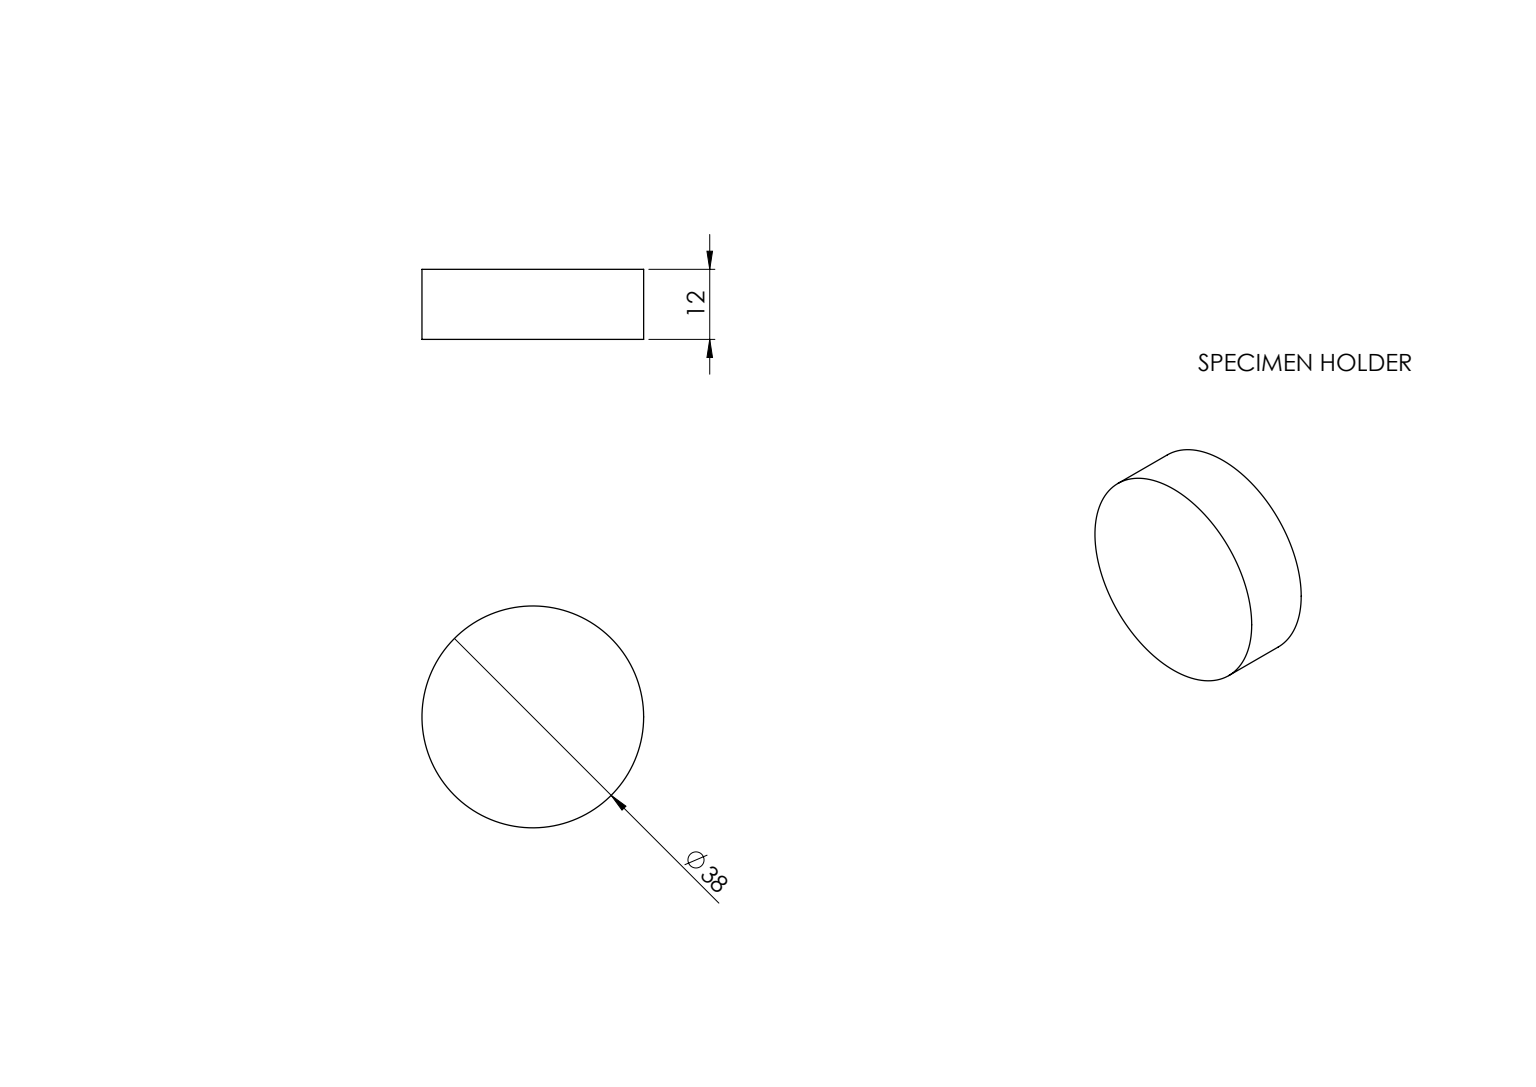
ISO-10303-21;
HEADER;
FILE_DESCRIPTION (('STEP AP214'),
    '1' );
FILE_NAME ('specimen holder.step',
    '2026-10-24T08:20:21',
    ( '' ),
    ( '' ),
    'SwSTEP 2.0',
    'SolidWorks 2026',
    '' );
FILE_SCHEMA (( 'AUTOMOTIVE_DESIGN' ));
ENDSEC;

DATA;
#4=DIRECTION ( 'NONE',  ( -0.000000000000000000, -0.000000000000000000, -1.000000000000000000 ) ) ;
#6=CARTESIAN_POINT ( 'NONE',  ( 0.000000000000000000, 0.000000000000000000, -15.70000000000000284 ) ) ;
#10=ORIENTED_EDGE ( 'NONE', *, *, #2629, .T. ) ;
#15=VERTEX_POINT ( 'NONE', #148 ) ;
#20=AXIS2_PLACEMENT_3D ( 'NONE', #499, #4, #521 ) ;
#29=VECTOR ( 'NONE', #2095, 1000.000000000000000 ) ;
#32=LINE ( 'NONE', #599, #2631 ) ;
#41=PRODUCT_DEFINITION_SHAPE ( 'NONE', 'NONE',  #583 ) ;
#63=ORIENTED_EDGE ( 'NONE', *, *, #1690, .T. ) ;
#78=EDGE_CURVE ( 'NONE', #2558, #3229, #1744, .T. ) ;
#89=CARTESIAN_POINT ( 'NONE',  ( 0.000000000000000000, 0.000000000000000000, -15.70000000000000284 ) ) ;
#97=ORIENTED_EDGE ( 'NONE', *, *, #3095, .F. ) ;
#110=ADVANCED_FACE ( 'NONE', ( #3446, #2287 ), #2899, .F. ) ;
#111=DIRECTION ( 'NONE',  ( -0.000000000000000000, -0.000000000000000000, -1.000000000000000000 ) ) ;
#148=CARTESIAN_POINT ( 'NONE',  ( -1.649999999999999911, 0.000000000000000000, -15.70000000000000284 ) ) ;
#167=ORIENTED_EDGE ( 'NONE', *, *, #1783, .T. ) ;
#177=ADVANCED_FACE ( 'NONE', ( #484 ), #3479, .T. ) ;
#181=FACE_OUTER_BOUND ( 'NONE', #2792, .T. ) ;
#199=PRODUCT_DEFINITION_CONTEXT ( 'detailed design', #1821, 'design' ) ;
#200=DIRECTION ( 'NONE',  ( 0.000000000000000000, 0.000000000000000000, 1.000000000000000000 ) ) ;
#203=MECHANICAL_DESIGN_GEOMETRIC_PRESENTATION_REPRESENTATION('',(#1878),#378);
#213=AXIS2_PLACEMENT_3D ( 'NONE', #1985, #1430, #779 ) ;
#251=CIRCLE ( 'NONE', #760, 18.99999999999999645 ) ;
#263=AXIS2_PLACEMENT_3D ( 'NONE', #1547, #656, #1261 ) ;
#268=( LENGTH_UNIT ( ) NAMED_UNIT ( * ) SI_UNIT ( .MILLI., .METRE. ) );
#280=DIRECTION ( 'NONE',  ( -0.000000000000000000, -0.000000000000000000, -1.000000000000000000 ) ) ;
#286=FACE_OUTER_BOUND ( 'NONE', #2486, .T. ) ;
#345=DIRECTION ( 'NONE',  ( 0.000000000000000000, 0.000000000000000000, 1.000000000000000000 ) ) ;
#348=DIRECTION ( 'NONE',  ( -0.000000000000000000, -0.000000000000000000, -1.000000000000000000 ) ) ;
#370=EDGE_LOOP ( 'NONE', ( #10, #1130 ) ) ;
#378=( GEOMETRIC_REPRESENTATION_CONTEXT ( 3 ) GLOBAL_UNCERTAINTY_ASSIGNED_CONTEXT ( ( #3167 ) ) GLOBAL_UNIT_ASSIGNED_CONTEXT ( ( #1308, #1913, #2493 ) ) REPRESENTATION_CONTEXT ( 'NONE', 'WORKASPACE' ) );
#387=DIRECTION ( 'NONE',  ( -0.000000000000000000, -0.000000000000000000, -1.000000000000000000 ) ) ;
#412=LINE ( 'NONE', #3056, #2644 ) ;
#418=APPLICATION_CONTEXT ( 'automotive_design' ) ;
#427=VERTEX_POINT ( 'NONE', #2778 ) ;
#432=DIRECTION ( 'NONE',  ( -0.000000000000000000, -0.000000000000000000, -1.000000000000000000 ) ) ;
#437=EDGE_CURVE ( 'NONE', #427, #715, #600, .T. ) ;
#445=ORIENTED_EDGE ( 'NONE', *, *, #866, .T. ) ;
#448=CARTESIAN_POINT ( 'NONE',  ( 0.000000000000000000, 0.000000000000000000, -15.70000000000000284 ) ) ;
#461=EDGE_CURVE ( 'NONE', #2373, #2385, #1905, .T. ) ;
#479=ORIENTED_EDGE ( 'NONE', *, *, #638, .F. ) ;
#481=DIRECTION ( 'NONE',  ( 0.000000000000000000, 0.000000000000000000, 1.000000000000000000 ) ) ;
#484=FACE_OUTER_BOUND ( 'NONE', #2820, .T. ) ;
#485=DIRECTION ( 'NONE',  ( -0.000000000000000000, -0.000000000000000000, -1.000000000000000000 ) ) ;
#499=CARTESIAN_POINT ( 'NONE',  ( 0.000000000000000000, 0.000000000000000000, -8.000000000000000000 ) ) ;
#510=DIRECTION ( 'NONE',  ( -0.000000000000000000, -0.000000000000000000, -1.000000000000000000 ) ) ;
#514=AXIS2_PLACEMENT_3D ( 'NONE', #1091, #878, #2301 ) ;
#521=DIRECTION ( 'NONE',  ( -1.000000000000000000, 0.000000000000000000, 0.000000000000000000 ) ) ;
#533=PRODUCT_DEFINITION_FORMATION_WITH_SPECIFIED_SOURCE ( 'ANY', '', #1906, .NOT_KNOWN. ) ;
#544=CARTESIAN_POINT ( 'NONE',  ( 0.000000000000000000, 0.000000000000000000, -8.000000000000000000 ) ) ;
#545=FILL_AREA_STYLE ('',( #2106 ) ) ;
#551=FACE_OUTER_BOUND ( 'NONE', #1433, .T. ) ;
#574=CARTESIAN_POINT ( 'NONE',  ( 0.000000000000000000, 0.000000000000000000, -14.99999999999999645 ) ) ;
#579=ORIENTED_EDGE ( 'NONE', *, *, #2275, .F. ) ;
#583=PRODUCT_DEFINITION ( 'UNKNOWN', '', #533, #199 ) ;
#592=ORIENTED_EDGE ( 'NONE', *, *, #78, .T. ) ;
#594=ORIENTED_EDGE ( 'NONE', *, *, #638, .T. ) ;
#599=CARTESIAN_POINT ( 'NONE',  ( -1.999999999999999112, 0.000000000000000000, -20.00000000000000000 ) ) ;
#600=CIRCLE ( 'NONE', #3082, 1.999999999999998224 ) ;
#611=VERTEX_POINT ( 'NONE', #2374 ) ;
#629=CARTESIAN_POINT ( 'NONE',  ( 0.000000000000000000, 0.000000000000000000, -20.00000000000000000 ) ) ;
#638=EDGE_CURVE ( 'NONE', #15, #2226, #783, .T. ) ;
#656=DIRECTION ( 'NONE',  ( 0.000000000000000000, 0.000000000000000000, 1.000000000000000000 ) ) ;
#674=DIRECTION ( 'NONE',  ( 0.8571673007021117785, 1.049727191138617956E-16, -0.5150380749100550437 ) ) ;
#682=DIRECTION ( 'NONE',  ( -1.000000000000000000, 0.000000000000000000, 0.000000000000000000 ) ) ;
#715=VERTEX_POINT ( 'NONE', #2469 ) ;
#760=AXIS2_PLACEMENT_3D ( 'NONE', #544, #883, #2067 ) ;
#767=CARTESIAN_POINT ( 'NONE',  ( -1.649999999999999245, 0.000000000000000000, -20.00000000000000000 ) ) ;
#770=AXIS2_PLACEMENT_3D ( 'NONE', #3342, #3320, #1841 ) ;
#771=AXIS2_PLACEMENT_3D ( 'NONE', #1959, #2015, #3203 ) ;
#775=DIRECTION ( 'NONE',  ( 1.000000000000000000, 0.000000000000000000, 0.000000000000000000 ) ) ;
#776=ADVANCED_FACE ( 'NONE', ( #1341 ), #3638, .F. ) ;
#779=DIRECTION ( 'NONE',  ( 1.000000000000000000, 0.000000000000000000, -0.000000000000000000 ) ) ;
#783=CIRCLE ( 'NONE', #3389, 1.649999999999999911 ) ;
#784=PRODUCT_CONTEXT ( 'NONE', #418, 'mechanical' ) ;
#797=DIRECTION ( 'NONE',  ( 0.000000000000000000, 0.000000000000000000, 1.000000000000000000 ) ) ;
#805=ORIENTED_EDGE ( 'NONE', *, *, #3212, .T. ) ;
#816=CARTESIAN_POINT ( 'NONE',  ( 0.000000000000000000, 0.000000000000000000, -8.000000000000000000 ) ) ;
#820=CARTESIAN_POINT ( 'NONE',  ( 0.000000000000000000, 0.000000000000000000, 0.000000000000000000 ) ) ;
#842=LINE ( 'NONE', #2086, #1695 ) ;
#843=PRESENTATION_STYLE_ASSIGNMENT (( #2655 ) ) ;
#863=DIRECTION ( 'NONE',  ( -1.000000000000000000, 0.000000000000000000, 0.000000000000000000 ) ) ;
#866=EDGE_CURVE ( 'NONE', #2558, #1368, #412, .T. ) ;
#875=DIRECTION ( 'NONE',  ( 1.000000000000000000, 0.000000000000000000, 0.000000000000000000 ) ) ;
#877=FACE_OUTER_BOUND ( 'NONE', #3535, .T. ) ;
#878=DIRECTION ( 'NONE',  ( -0.000000000000000000, -0.000000000000000000, -1.000000000000000000 ) ) ;
#883=DIRECTION ( 'NONE',  ( 0.000000000000000000, 0.000000000000000000, 1.000000000000000000 ) ) ;
#884=( LENGTH_UNIT ( ) NAMED_UNIT ( * ) SI_UNIT ( .MILLI., .METRE. ) );
#908=( GEOMETRIC_REPRESENTATION_CONTEXT ( 3 ) GLOBAL_UNCERTAINTY_ASSIGNED_CONTEXT ( ( #3619 ) ) GLOBAL_UNIT_ASSIGNED_CONTEXT ( ( #884, #1793, #924 ) ) REPRESENTATION_CONTEXT ( 'NONE', 'WORKASPACE' ) );
#921=ORIENTED_EDGE ( 'NONE', *, *, #437, .T. ) ;
#924=( NAMED_UNIT ( * ) SI_UNIT ( $, .STERADIAN. ) SOLID_ANGLE_UNIT ( ) );
#928=CARTESIAN_POINT ( 'NONE',  ( -1.649999999999998579, 0.000000000000000000, -14.99999999999999645 ) ) ;
#957=DIRECTION ( 'NONE',  ( -0.000000000000000000, -0.000000000000000000, -1.000000000000000000 ) ) ;
#961=SHAPE_REPRESENTATION ( 'specimen holder', ( #2207 ), #908 ) ;
#978=CARTESIAN_POINT ( 'NONE',  ( 0.000000000000000000, 0.000000000000000000, -20.00000000000000000 ) ) ;
#979=CARTESIAN_POINT ( 'NONE',  ( 1.999999999999999112, 2.449293598294705428E-16, -20.00000000000000000 ) ) ;
#992=DIRECTION ( 'NONE',  ( -0.000000000000000000, -0.000000000000000000, -1.000000000000000000 ) ) ;
#1030=ORIENTED_EDGE ( 'NONE', *, *, #3165, .T. ) ;
#1033=DIRECTION ( 'NONE',  ( -0.000000000000000000, -0.000000000000000000, -1.000000000000000000 ) ) ;
#1056=DIRECTION ( 'NONE',  ( -1.000000000000000000, 0.000000000000000000, 0.000000000000000000 ) ) ;
#1067=CARTESIAN_POINT ( 'NONE',  ( 0.000000000000000000, 0.000000000000000000, -14.99999999999999645 ) ) ;
#1089=EDGE_LOOP ( 'NONE', ( #2639, #1113, #2464, #921 ) ) ;
#1091=CARTESIAN_POINT ( 'NONE',  ( 0.000000000000000000, 0.000000000000000000, -15.70000000000000284 ) ) ;
#1105=VERTEX_POINT ( 'NONE', #2333 ) ;
#1113=ORIENTED_EDGE ( 'NONE', *, *, #2629, .F. ) ;
#1130=ORIENTED_EDGE ( 'NONE', *, *, #461, .T. ) ;
#1144=ADVANCED_FACE ( 'NONE', ( #3825 ), #2279, .T. ) ;
#1176=ORIENTED_EDGE ( 'NONE', *, *, #437, .F. ) ;
#1181=DIRECTION ( 'NONE',  ( -0.000000000000000000, -0.000000000000000000, -1.000000000000000000 ) ) ;
#1229=CLOSED_SHELL ( 'NONE', ( #776, #1258, #1235, #177, #1944, #1144, #2674, #3048, #1994, #110, #2461 ) ) ;
#1230=DIRECTION ( 'NONE',  ( -1.000000000000000000, 0.000000000000000000, 0.000000000000000000 ) ) ;
#1235=ADVANCED_FACE ( 'NONE', ( #877 ), #2964, .F. ) ;
#1239=DIRECTION ( 'NONE',  ( -1.000000000000000000, 0.000000000000000000, 0.000000000000000000 ) ) ;
#1258=ADVANCED_FACE ( 'NONE', ( #2744 ), #1594, .F. ) ;
#1261=DIRECTION ( 'NONE',  ( 1.000000000000000000, 0.000000000000000000, -0.000000000000000000 ) ) ;
#1274=EDGE_CURVE ( 'NONE', #2771, #611, #3236, .T. ) ;
#1308=( LENGTH_UNIT ( ) NAMED_UNIT ( * ) SI_UNIT ( .MILLI., .METRE. ) );
#1318=ORIENTED_EDGE ( 'NONE', *, *, #3095, .T. ) ;
#1341=FACE_OUTER_BOUND ( 'NONE', #3463, .T. ) ;
#1368=VERTEX_POINT ( 'NONE', #2293 ) ;
#1370=PLANE ( 'NONE',  #263 ) ;
#1387=CIRCLE ( 'NONE', #3557, 18.99999999999999645 ) ;
#1393=CIRCLE ( 'NONE', #2132, 2.000000000000000000 ) ;
#1394=DIRECTION ( 'NONE',  ( 1.000000000000000000, 0.000000000000000000, 0.000000000000000000 ) ) ;
#1418=ORIENTED_EDGE ( 'NONE', *, *, #2998, .T. ) ;
#1430=DIRECTION ( 'NONE',  ( 0.000000000000000000, 0.000000000000000000, 1.000000000000000000 ) ) ;
#1433=EDGE_LOOP ( 'NONE', ( #2166, #592, #1418 ) ) ;
#1442=EDGE_LOOP ( 'NONE', ( #1318, #2099 ) ) ;
#1448=CIRCLE ( 'NONE', #3371, 18.99999999999999645 ) ;
#1489=EDGE_CURVE ( 'NONE', #1105, #3089, #842, .T. ) ;
#1497=ORIENTED_EDGE ( 'NONE', *, *, #3426, .F. ) ;
#1503=CIRCLE ( 'NONE', #2570, 18.99999999999999645 ) ;
#1507=DIRECTION ( 'NONE',  ( -0.000000000000000000, -0.000000000000000000, -1.000000000000000000 ) ) ;
#1533=EDGE_CURVE ( 'NONE', #2771, #1105, #251, .T. ) ;
#1547=CARTESIAN_POINT ( 'NONE',  ( 0.000000000000000000, 0.000000000000000000, -20.00000000000000000 ) ) ;
#1549=DIRECTION ( 'NONE',  ( -1.000000000000000000, 0.000000000000000000, 0.000000000000000000 ) ) ;
#1580=DIRECTION ( 'NONE',  ( -1.000000000000000000, 0.000000000000000000, 0.000000000000000000 ) ) ;
#1594=CYLINDRICAL_SURFACE ( 'NONE', #1652, 1.649999999999999245 ) ;
#1611=SHAPE_DEFINITION_REPRESENTATION ( #41, #961 ) ;
#1625=CIRCLE ( 'NONE', #3802, 1.649999999999998579 ) ;
#1652=AXIS2_PLACEMENT_3D ( 'NONE', #2785, #111, #2351 ) ;
#1690=EDGE_CURVE ( 'NONE', #2373, #715, #3622, .T. ) ;
#1695=VECTOR ( 'NONE', #3815, 1000.000000000000000 ) ;
#1735=SURFACE_SIDE_STYLE ('',( #3799 ) ) ;
#1744=LINE ( 'NONE', #2916, #2484 ) ;
#1762=CARTESIAN_POINT ( 'NONE',  ( 18.99999999999999645, 2.326828918379970576E-15, -8.000000000000000000 ) ) ;
#1765=CIRCLE ( 'NONE', #2574, 1.649999999999998579 ) ;
#1783=EDGE_CURVE ( 'NONE', #1368, #3229, #1625, .T. ) ;
#1793=( NAMED_UNIT ( * ) PLANE_ANGLE_UNIT ( ) SI_UNIT ( $, .RADIAN. ) );
#1797=ORIENTED_EDGE ( 'NONE', *, *, #461, .F. ) ;
#1821=APPLICATION_CONTEXT ( 'automotive_design' ) ;
#1841=DIRECTION ( 'NONE',  ( -1.000000000000000000, 0.000000000000000000, 0.000000000000000000 ) ) ;
#1845=CARTESIAN_POINT ( 'NONE',  ( 0.000000000000000000, 0.000000000000000000, -20.00000000000000000 ) ) ;
#1878=STYLED_ITEM('',(#3888),#3238);
#1894=COLOUR_RGB ( '',0.8941176470588234615, 0.8941176470588234615, 0.8941176470588234615 ) ;
#1905=CIRCLE ( 'NONE', #3773, 2.000000000000000000 ) ;
#1906=PRODUCT ( 'specimen holder', 'specimen holder', '', ( #784 ) ) ;
#1913=( NAMED_UNIT ( * ) PLANE_ANGLE_UNIT ( ) SI_UNIT ( $, .RADIAN. ) );
#1934=ORIENTED_EDGE ( 'NONE', *, *, #2178, .T. ) ;
#1944=ADVANCED_FACE ( 'NONE', ( #286 ), #2669, .T. ) ;
#1956=ORIENTED_EDGE ( 'NONE', *, *, #2275, .T. ) ;
#1959=CARTESIAN_POINT ( 'NONE',  ( 0.000000000000000000, 0.000000000000000000, -14.99999999999999645 ) ) ;
#1985=CARTESIAN_POINT ( 'NONE',  ( 1.649999999999999911, 0.000000000000000000, -15.70000000000000284 ) ) ;
#1994=ADVANCED_FACE ( 'NONE', ( #3635 ), #3325, .F. ) ;
#2002=DIRECTION ( 'NONE',  ( -0.000000000000000000, -0.000000000000000000, -1.000000000000000000 ) ) ;
#2008=VECTOR ( 'NONE', #3163, 1000.000000000000000 ) ;
#2015=DIRECTION ( 'NONE',  ( -0.000000000000000000, -0.000000000000000000, -1.000000000000000000 ) ) ;
#2055=ORIENTED_EDGE ( 'NONE', *, *, #1274, .F. ) ;
#2067=DIRECTION ( 'NONE',  ( 1.000000000000000000, 0.000000000000000000, 0.000000000000000000 ) ) ;
#2078=CARTESIAN_POINT ( 'NONE',  ( 2.000000000000000000, 2.449293598294706414E-16, -15.70000000000000284 ) ) ;
#2085=DIRECTION ( 'NONE',  ( -0.000000000000000000, -0.000000000000000000, -1.000000000000000000 ) ) ;
#2086=CARTESIAN_POINT ( 'NONE',  ( -18.99999999999999645, 0.000000000000000000, -8.000000000000000000 ) ) ;
#2087=( NAMED_UNIT ( * ) PLANE_ANGLE_UNIT ( ) SI_UNIT ( $, .RADIAN. ) );
#2095=DIRECTION ( 'NONE',  ( -0.000000000000000000, -0.000000000000000000, -1.000000000000000000 ) ) ;
#2099=ORIENTED_EDGE ( 'NONE', *, *, #1533, .T. ) ;
#2106=FILL_AREA_STYLE_COLOUR ( '', #1894 ) ;
#2126=CARTESIAN_POINT ( 'NONE',  ( 1.649999999999999245, 2.020667218593132015E-16, -20.00000000000000000 ) ) ;
#2130=CIRCLE ( 'NONE', #2628, 1.999999999999998224 ) ;
#2132=AXIS2_PLACEMENT_3D ( 'NONE', #448, #387, #1580 ) ;
#2141=STYLED_ITEM ( 'NONE', ( #843 ), #2739 ) ;
#2166=ORIENTED_EDGE ( 'NONE', *, *, #866, .F. ) ;
#2178=EDGE_CURVE ( 'NONE', #611, #3089, #1503, .T. ) ;
#2188=ORIENTED_EDGE ( 'NONE', *, *, #1533, .F. ) ;
#2205=EDGE_LOOP ( 'NONE', ( #479, #579 ) ) ;
#2207=AXIS2_PLACEMENT_3D ( 'NONE', #820, #2246, #3194 ) ;
#2226=VERTEX_POINT ( 'NONE', #2483 ) ;
#2246=DIRECTION ( 'NONE',  ( 0.000000000000000000, 0.000000000000000000, 1.000000000000000000 ) ) ;
#2275=EDGE_CURVE ( 'NONE', #2226, #15, #2504, .T. ) ;
#2276=UNCERTAINTY_MEASURE_WITH_UNIT (LENGTH_MEASURE( 1.000000000000000082E-05 ), #268, 'distance_accuracy_value', 'NONE');
#2279=PLANE ( 'NONE',  #2586 ) ;
#2287=FACE_OUTER_BOUND ( 'NONE', #370, .T. ) ;
#2293=CARTESIAN_POINT ( 'NONE',  ( 1.649999999999998579, 2.020667218593131029E-16, -14.99999999999999645 ) ) ;
#2301=DIRECTION ( 'NONE',  ( -1.000000000000000000, 0.000000000000000000, 0.000000000000000000 ) ) ;
#2333=CARTESIAN_POINT ( 'NONE',  ( -18.99999999999999645, 0.000000000000000000, -8.000000000000000000 ) ) ;
#2351=DIRECTION ( 'NONE',  ( -1.000000000000000000, 0.000000000000000000, 0.000000000000000000 ) ) ;
#2353=EDGE_CURVE ( 'NONE', #715, #427, #2130, .T. ) ;
#2355=ORIENTED_EDGE ( 'NONE', *, *, #1274, .T. ) ;
#2364=ORIENTED_EDGE ( 'NONE', *, *, #1489, .F. ) ;
#2373=VERTEX_POINT ( 'NONE', #2078 ) ;
#2374=CARTESIAN_POINT ( 'NONE',  ( 18.99999999999999645, 2.326828918379970576E-15, -20.00000000000000000 ) ) ;
#2385=VERTEX_POINT ( 'NONE', #3296 ) ;
#2400=SHAPE_REPRESENTATION_RELATIONSHIP ( 'NONE' , 'NONE' ,  #961, #2739 ) ;
#2411=CARTESIAN_POINT ( 'NONE',  ( 18.99999999999999645, 2.326828918379970576E-15, -8.000000000000000000 ) ) ;
#2461=ADVANCED_FACE ( 'NONE', ( #3259 ), #3013, .F. ) ;
#2464=ORIENTED_EDGE ( 'NONE', *, *, #2468, .T. ) ;
#2468=EDGE_CURVE ( 'NONE', #2385, #427, #32, .T. ) ;
#2469=CARTESIAN_POINT ( 'NONE',  ( 1.999999999999998224, 2.449293598294704935E-16, -20.00000000000000355 ) ) ;
#2483=CARTESIAN_POINT ( 'NONE',  ( 1.649999999999999911, 2.020667218593133001E-16, -15.70000000000000284 ) ) ;
#2484=VECTOR ( 'NONE', #2567, 1000.000000000000000 ) ;
#2486=EDGE_LOOP ( 'NONE', ( #2055, #97, #3119, #805 ) ) ;
#2493=( NAMED_UNIT ( * ) SI_UNIT ( $, .STERADIAN. ) SOLID_ANGLE_UNIT ( ) );
#2495=CARTESIAN_POINT ( 'NONE',  ( -1.467474670309871178E-15, 0.000000000000000000, -14.00857997860452109 ) ) ;
#2498=ORIENTED_EDGE ( 'NONE', *, *, #2178, .F. ) ;
#2504=CIRCLE ( 'NONE', #514, 1.649999999999999911 ) ;
#2517=ORIENTED_EDGE ( 'NONE', *, *, #2998, .F. ) ;
#2534=CARTESIAN_POINT ( 'NONE',  ( 0.000000000000000000, 0.000000000000000000, -14.99999999999999645 ) ) ;
#2552=DIRECTION ( 'NONE',  ( -1.000000000000000000, 0.000000000000000000, 0.000000000000000000 ) ) ;
#2558=VERTEX_POINT ( 'NONE', #2495 ) ;
#2567=DIRECTION ( 'NONE',  ( -0.8571673007021117785, 0.000000000000000000, -0.5150380749100550437 ) ) ;
#2570=AXIS2_PLACEMENT_3D ( 'NONE', #3155, #481, #775 ) ;
#2574=AXIS2_PLACEMENT_3D ( 'NONE', #1067, #510, #2613 ) ;
#2577=AXIS2_PLACEMENT_3D ( 'NONE', #816, #2002, #863 ) ;
#2586=AXIS2_PLACEMENT_3D ( 'NONE', #3464, #797, #3776 ) ;
#2613=DIRECTION ( 'NONE',  ( -1.000000000000000000, 0.000000000000000000, 0.000000000000000000 ) ) ;
#2625=EDGE_LOOP ( 'NONE', ( #1176, #3590 ) ) ;
#2628=AXIS2_PLACEMENT_3D ( 'NONE', #3549, #1181, #1239 ) ;
#2629=EDGE_CURVE ( 'NONE', #2385, #2373, #1393, .T. ) ;
#2631=VECTOR ( 'NONE', #280, 1000.000000000000000 ) ;
#2639=ORIENTED_EDGE ( 'NONE', *, *, #1690, .F. ) ;
#2644=VECTOR ( 'NONE', #674, 1000.000000000000000 ) ;
#2655=SURFACE_STYLE_USAGE ( .BOTH. , #1735 ) ;
#2669=CYLINDRICAL_SURFACE ( 'NONE', #20, 18.99999999999999645 ) ;
#2674=ADVANCED_FACE ( 'NONE', ( #2853, #181 ), #1370, .F. ) ;
#2697=LINE ( 'NONE', #2126, #29 ) ;
#2739=ADVANCED_BREP_SHAPE_REPRESENTATION ( '', ( #3238, #2207 ), #908 ) ;
#2744=FACE_OUTER_BOUND ( 'NONE', #3527, .T. ) ;
#2771=VERTEX_POINT ( 'NONE', #2411 ) ;
#2778=CARTESIAN_POINT ( 'NONE',  ( -1.999999999999998224, 0.000000000000000000, -20.00000000000000355 ) ) ;
#2780=DIRECTION ( 'NONE',  ( -1.000000000000000000, 0.000000000000000000, 0.000000000000000000 ) ) ;
#2785=CARTESIAN_POINT ( 'NONE',  ( 0.000000000000000000, 0.000000000000000000, -20.00000000000000000 ) ) ;
#2792=EDGE_LOOP ( 'NONE', ( #3340, #2498 ) ) ;
#2794=DIRECTION ( 'NONE',  ( -1.000000000000000000, 0.000000000000000000, 0.000000000000000000 ) ) ;
#2804=ORIENTED_EDGE ( 'NONE', *, *, #3426, .T. ) ;
#2820=EDGE_LOOP ( 'NONE', ( #2188, #2355, #1934, #2364 ) ) ;
#2826=MECHANICAL_DESIGN_GEOMETRIC_PRESENTATION_REPRESENTATION('',(#2141),#3144);
#2827=AXIS2_PLACEMENT_3D ( 'NONE', #978, #432, #2780 ) ;
#2853=FACE_BOUND ( 'NONE', #2625, .T. ) ;
#2866=CARTESIAN_POINT ( 'NONE',  ( 0.000000000000000000, 0.000000000000000000, -8.000000000000000000 ) ) ;
#2899=PLANE ( 'NONE',  #213 ) ;
#2916=CARTESIAN_POINT ( 'NONE',  ( -1.649999999999998579, 0.000000000000000000, -14.99999999999999645 ) ) ;
#2953=DIRECTION ( 'NONE',  ( -0.000000000000000000, -0.000000000000000000, -1.000000000000000000 ) ) ;
#2964=CONICAL_SURFACE ( 'NONE', #3267, 1.649999999999998579, 1.029744258676653423 ) ;
#2975=EDGE_LOOP ( 'NONE', ( #3352, #2517, #2804, #594 ) ) ;
#2998=EDGE_CURVE ( 'NONE', #3229, #1368, #1765, .T. ) ;
#3013=CYLINDRICAL_SURFACE ( 'NONE', #770, 1.999999999999999112 ) ;
#3039=CARTESIAN_POINT ( 'NONE',  ( 0.000000000000000000, 0.000000000000000000, -20.00000000000000355 ) ) ;
#3048=ADVANCED_FACE ( 'NONE', ( #551 ), #3694, .F. ) ;
#3056=CARTESIAN_POINT ( 'NONE',  ( 1.649999999999998579, 2.020667218593131029E-16, -14.99999999999999645 ) ) ;
#3082=AXIS2_PLACEMENT_3D ( 'NONE', #3039, #992, #2794 ) ;
#3089=VERTEX_POINT ( 'NONE', #3473 ) ;
#3095=EDGE_CURVE ( 'NONE', #1105, #2771, #1387, .T. ) ;
#3112=ORIENTED_EDGE ( 'NONE', *, *, #2468, .F. ) ;
#3119=ORIENTED_EDGE ( 'NONE', *, *, #1489, .T. ) ;
#3138=ORIENTED_EDGE ( 'NONE', *, *, #78, .F. ) ;
#3144=( GEOMETRIC_REPRESENTATION_CONTEXT ( 3 ) GLOBAL_UNCERTAINTY_ASSIGNED_CONTEXT ( ( #2276 ) ) GLOBAL_UNIT_ASSIGNED_CONTEXT ( ( #268, #2087, #3525 ) ) REPRESENTATION_CONTEXT ( 'NONE', 'WORKASPACE' ) );
#3155=CARTESIAN_POINT ( 'NONE',  ( 0.000000000000000000, 0.000000000000000000, -20.00000000000000000 ) ) ;
#3163=DIRECTION ( 'NONE',  ( -0.000000000000000000, -0.000000000000000000, -1.000000000000000000 ) ) ;
#3165=EDGE_CURVE ( 'NONE', #1368, #2226, #2697, .T. ) ;
#3167=UNCERTAINTY_MEASURE_WITH_UNIT (LENGTH_MEASURE( 1.000000000000000082E-05 ), #1308, 'distance_accuracy_value', 'NONE');
#3194=DIRECTION ( 'NONE',  ( 1.000000000000000000, 0.000000000000000000, 0.000000000000000000 ) ) ;
#3203=DIRECTION ( 'NONE',  ( -1.000000000000000000, 0.000000000000000000, 0.000000000000000000 ) ) ;
#3212=EDGE_CURVE ( 'NONE', #3089, #611, #1448, .T. ) ;
#3229=VERTEX_POINT ( 'NONE', #928 ) ;
#3236=LINE ( 'NONE', #1762, #3583 ) ;
#3238=MANIFOLD_SOLID_BREP ( 'M4 Tapped Hole1', #1229 ) ;
#3259=FACE_OUTER_BOUND ( 'NONE', #1089, .T. ) ;
#3267=AXIS2_PLACEMENT_3D ( 'NONE', #574, #348, #682 ) ;
#3296=CARTESIAN_POINT ( 'NONE',  ( -2.000000000000000000, 0.000000000000000000, -15.70000000000000284 ) ) ;
#3320=DIRECTION ( 'NONE',  ( -0.000000000000000000, -0.000000000000000000, -1.000000000000000000 ) ) ;
#3325=CYLINDRICAL_SURFACE ( 'NONE', #3623, 1.649999999999999245 ) ;
#3340=ORIENTED_EDGE ( 'NONE', *, *, #3212, .F. ) ;
#3342=CARTESIAN_POINT ( 'NONE',  ( 0.000000000000000000, 0.000000000000000000, -20.00000000000000000 ) ) ;
#3352=ORIENTED_EDGE ( 'NONE', *, *, #3165, .F. ) ;
#3371=AXIS2_PLACEMENT_3D ( 'NONE', #629, #345, #875 ) ;
#3389=AXIS2_PLACEMENT_3D ( 'NONE', #6, #2085, #1230 ) ;
#3426=EDGE_CURVE ( 'NONE', #3229, #15, #3432, .T. ) ;
#3432=LINE ( 'NONE', #767, #2008 ) ;
#3446=FACE_BOUND ( 'NONE', #2205, .T. ) ;
#3457=ORIENTED_EDGE ( 'NONE', *, *, #1783, .F. ) ;
#3463=EDGE_LOOP ( 'NONE', ( #1797, #63, #3804, #3112 ) ) ;
#3464=CARTESIAN_POINT ( 'NONE',  ( 0.000000000000000000, 0.000000000000000000, -8.000000000000000000 ) ) ;
#3473=CARTESIAN_POINT ( 'NONE',  ( -18.99999999999999645, 0.000000000000000000, -20.00000000000000000 ) ) ;
#3479=CYLINDRICAL_SURFACE ( 'NONE', #2577, 18.99999999999999645 ) ;
#3525=( NAMED_UNIT ( * ) SI_UNIT ( $, .STERADIAN. ) SOLID_ANGLE_UNIT ( ) );
#3527=EDGE_LOOP ( 'NONE', ( #3457, #1030, #1956, #1497 ) ) ;
#3535=EDGE_LOOP ( 'NONE', ( #3138, #445, #167 ) ) ;
#3549=CARTESIAN_POINT ( 'NONE',  ( 0.000000000000000000, 0.000000000000000000, -20.00000000000000355 ) ) ;
#3553=VECTOR ( 'NONE', #957, 1000.000000000000000 ) ;
#3557=AXIS2_PLACEMENT_3D ( 'NONE', #2866, #200, #1394 ) ;
#3583=VECTOR ( 'NONE', #2953, 1000.000000000000000 ) ;
#3590=ORIENTED_EDGE ( 'NONE', *, *, #2353, .F. ) ;
#3619=UNCERTAINTY_MEASURE_WITH_UNIT (LENGTH_MEASURE( 1.000000000000000082E-05 ), #884, 'distance_accuracy_value', 'NONE');
#3622=LINE ( 'NONE', #979, #3553 ) ;
#3623=AXIS2_PLACEMENT_3D ( 'NONE', #1845, #1507, #1549 ) ;
#3635=FACE_OUTER_BOUND ( 'NONE', #2975, .T. ) ;
#3638=CYLINDRICAL_SURFACE ( 'NONE', #2827, 1.999999999999999112 ) ;
#3694=CONICAL_SURFACE ( 'NONE', #771, 1.649999999999998579, 1.029744258676653423 ) ;
#3773=AXIS2_PLACEMENT_3D ( 'NONE', #89, #1033, #1056 ) ;
#3776=DIRECTION ( 'NONE',  ( 1.000000000000000000, 0.000000000000000000, -0.000000000000000000 ) ) ;
#3799=SURFACE_STYLE_FILL_AREA ( #545 ) ;
#3802=AXIS2_PLACEMENT_3D ( 'NONE', #2534, #485, #2552 ) ;
#3804=ORIENTED_EDGE ( 'NONE', *, *, #2353, .T. ) ;
#3815=DIRECTION ( 'NONE',  ( -0.000000000000000000, -0.000000000000000000, -1.000000000000000000 ) ) ;
#3825=FACE_OUTER_BOUND ( 'NONE', #1442, .T. ) ;
#3882=COLOUR_RGB('Off White',0.89,0.88,0.83);
#3883=FILL_AREA_STYLE_COLOUR('',#3882);
#3884=FILL_AREA_STYLE('',(#3883));
#3885=SURFACE_STYLE_FILL_AREA(#3884);
#3886=SURFACE_SIDE_STYLE('',(#3885));
#3887=SURFACE_STYLE_USAGE(.BOTH.,#3886);
#3888=PRESENTATION_STYLE_ASSIGNMENT((#3887));
ENDSEC;
END-ISO-10303-21;
